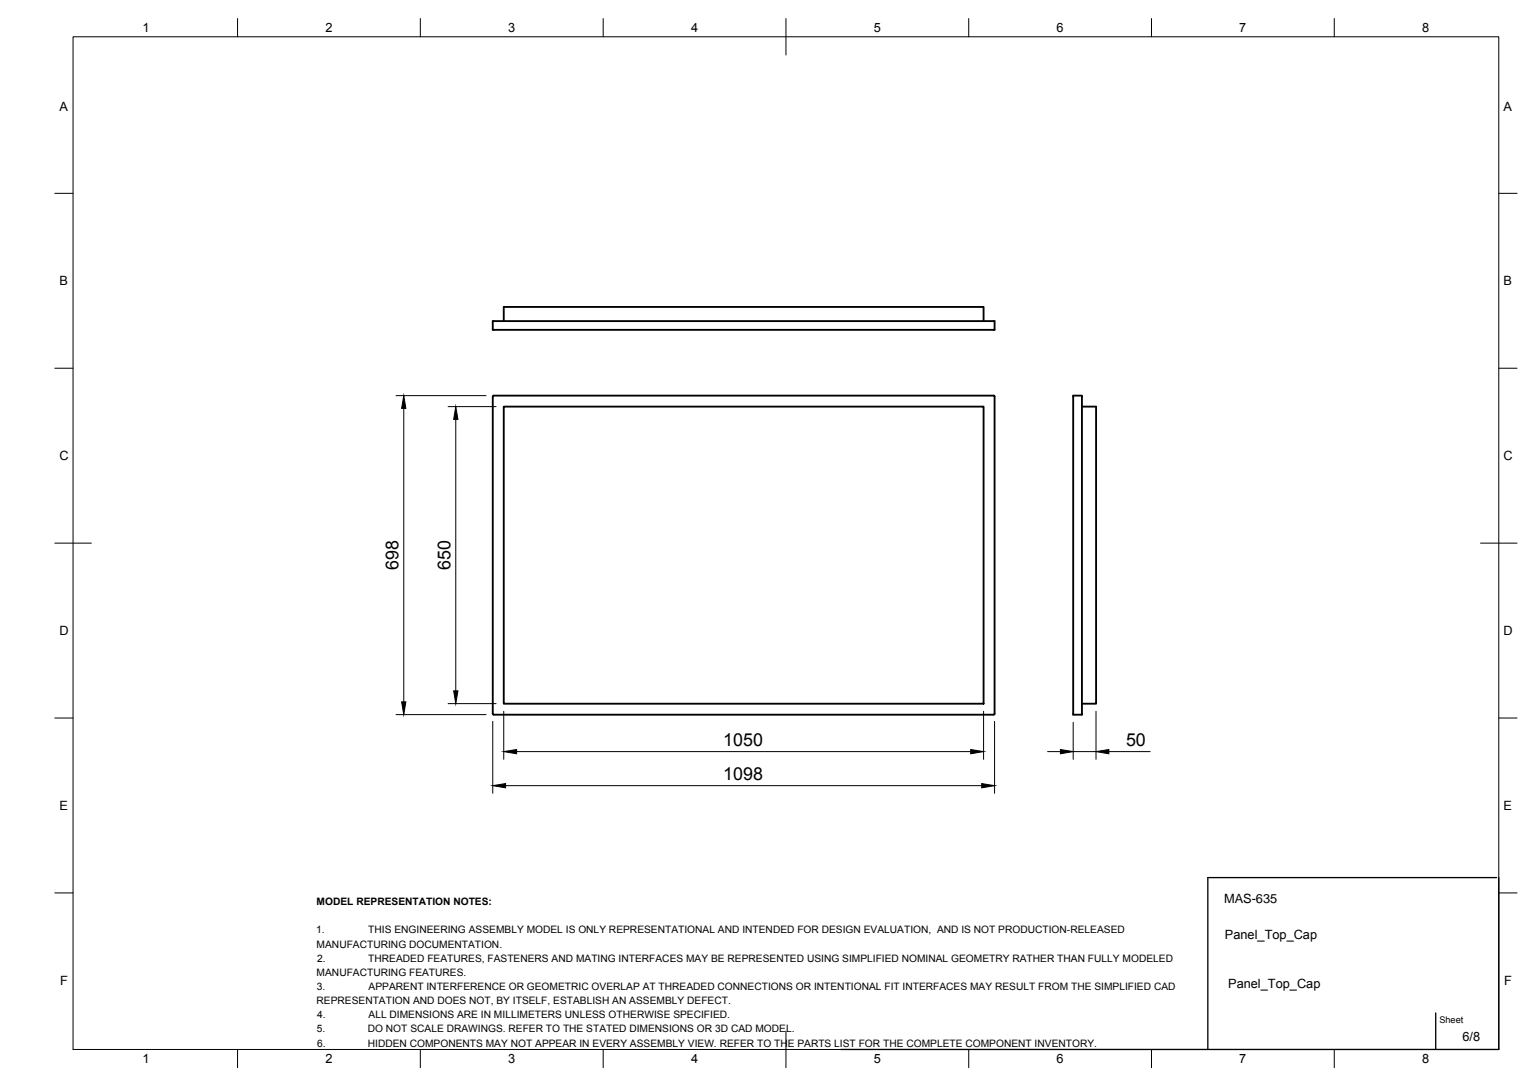
ISO-10303-21;
HEADER;
FILE_DESCRIPTION((''),'2;1');
FILE_NAME('Panel_Top_Cap.step','2026-10-09T12:34:24-07:00',(''),(''),'','','');
FILE_SCHEMA (('AUTOMOTIVE_DESIGN { 1 0 10303 214 3 1 1 }'));
ENDSEC;
DATA;
#10=MECHANICAL_DESIGN_GEOMETRIC_PRESENTATION_REPRESENTATION('',(#62),#3759);
#50=SHAPE_REPRESENTATION_RELATIONSHIP('SRR','None',#3791,#56) ;
#56=ADVANCED_BREP_SHAPE_REPRESENTATION('',(#68),#3756) ;
#62=STYLED_ITEM('',(#3827),#68) ;
#68=MANIFOLD_SOLID_BREP('Body1',#2266) ;
#83=CYLINDRICAL_SURFACE('',#2449,0.2) ;
#84=CYLINDRICAL_SURFACE('',#2450,0.2) ;
#85=CYLINDRICAL_SURFACE('',#2451,0.2) ;
#86=CYLINDRICAL_SURFACE('',#2452,0.2) ;
#111=CIRCLE('',#2440,0.2) ;
#112=CIRCLE('',#2441,0.2) ;
#113=CIRCLE('',#2442,0.2) ;
#114=CIRCLE('',#2443,0.2) ;
#115=CIRCLE('',#2445,0.2) ;
#116=CIRCLE('',#2446,0.2) ;
#117=CIRCLE('',#2447,0.2) ;
#118=CIRCLE('',#2448,0.2) ;
#132=FACE_BOUND('',#349,.T.) ;
#206=FACE_OUTER_BOUND('',#339,.T.) ;
#207=FACE_OUTER_BOUND('',#340,.T.) ;
#208=FACE_OUTER_BOUND('',#341,.T.) ;
#209=FACE_OUTER_BOUND('',#342,.T.) ;
#210=FACE_OUTER_BOUND('',#343,.T.) ;
#211=FACE_OUTER_BOUND('',#344,.T.) ;
#212=FACE_OUTER_BOUND('',#345,.T.) ;
#213=FACE_OUTER_BOUND('',#346,.T.) ;
#214=FACE_OUTER_BOUND('',#347,.T.) ;
#215=FACE_OUTER_BOUND('',#348,.T.) ;
#216=FACE_OUTER_BOUND('',#350,.T.) ;
#217=FACE_OUTER_BOUND('',#351,.T.) ;
#218=FACE_OUTER_BOUND('',#352,.T.) ;
#219=FACE_OUTER_BOUND('',#353,.T.) ;
#220=FACE_OUTER_BOUND('',#354,.T.) ;
#339=EDGE_LOOP('',(#1775,#1776,#1777,#1778)) ;
#340=EDGE_LOOP('',(#1779,#1780,#1781,#1782)) ;
#341=EDGE_LOOP('',(#1783,#1784,#1785,#1786)) ;
#342=EDGE_LOOP('',(#1787,#1788,#1789,#1790)) ;
#343=EDGE_LOOP('',(#1791,#1792,#1793,#1794)) ;
#344=EDGE_LOOP('',(#1795,#1796,#1797,#1798)) ;
#345=EDGE_LOOP('',(#1799,#1800,#1801,#1802)) ;
#346=EDGE_LOOP('',(#1803,#1804,#1805,#1806)) ;
#347=EDGE_LOOP('',(#1807,#1808,#1809,#1810)) ;
#348=EDGE_LOOP('',(#1811,#1812,#1813,#1814,#1815,#1816,#1817,#1818)) ;
#349=EDGE_LOOP('',(#1819,#1820,#1821,#1822)) ;
#350=EDGE_LOOP('',(#1823,#1824,#1825,#1826,#1827,#1828,#1829,#1830)) ;
#351=EDGE_LOOP('',(#1831,#1832,#1833,#1834)) ;
#352=EDGE_LOOP('',(#1835,#1836,#1837,#1838)) ;
#353=EDGE_LOOP('',(#1839,#1840,#1841,#1842)) ;
#354=EDGE_LOOP('',(#1843,#1844,#1845,#1846)) ;
#547=LINE('',#3461,#815) ;
#548=LINE('',#3463,#816) ;
#549=LINE('',#3465,#817) ;
#550=LINE('',#3466,#818) ;
#551=LINE('',#3469,#819) ;
#552=LINE('',#3471,#820) ;
#553=LINE('',#3472,#821) ;
#554=LINE('',#3475,#822) ;
#555=LINE('',#3477,#823) ;
#556=LINE('',#3478,#824) ;
#557=LINE('',#3480,#825) ;
#558=LINE('',#3481,#826) ;
#559=LINE('',#3486,#827) ;
#560=LINE('',#3488,#828) ;
#561=LINE('',#3490,#829) ;
#562=LINE('',#3491,#830) ;
#563=LINE('',#3495,#831) ;
#564=LINE('',#3497,#832) ;
#565=LINE('',#3499,#833) ;
#566=LINE('',#3500,#834) ;
#567=LINE('',#3504,#835) ;
#568=LINE('',#3506,#836) ;
#569=LINE('',#3508,#837) ;
#570=LINE('',#3509,#838) ;
#571=LINE('',#3513,#839) ;
#572=LINE('',#3515,#840) ;
#573=LINE('',#3517,#841) ;
#574=LINE('',#3518,#842) ;
#815=VECTOR('',#2838,100.) ;
#816=VECTOR('',#2839,100.) ;
#817=VECTOR('',#2840,100.) ;
#818=VECTOR('',#2841,100.) ;
#819=VECTOR('',#2844,100.) ;
#820=VECTOR('',#2845,100.) ;
#821=VECTOR('',#2846,100.) ;
#822=VECTOR('',#2849,100.) ;
#823=VECTOR('',#2850,100.) ;
#824=VECTOR('',#2851,100.) ;
#825=VECTOR('',#2854,100.) ;
#826=VECTOR('',#2855,100.) ;
#827=VECTOR('',#2860,100.) ;
#828=VECTOR('',#2861,100.) ;
#829=VECTOR('',#2862,100.) ;
#830=VECTOR('',#2863,100.) ;
#831=VECTOR('',#2866,100.) ;
#832=VECTOR('',#2867,100.) ;
#833=VECTOR('',#2868,100.) ;
#834=VECTOR('',#2869,100.) ;
#835=VECTOR('',#2872,100.) ;
#836=VECTOR('',#2873,100.) ;
#837=VECTOR('',#2874,100.) ;
#838=VECTOR('',#2875,100.) ;
#839=VECTOR('',#2878,100.) ;
#840=VECTOR('',#2879,100.) ;
#841=VECTOR('',#2880,100.) ;
#842=VECTOR('',#2881,100.) ;
#1051=VERTEX_POINT('',#3459) ;
#1052=VERTEX_POINT('',#3460) ;
#1053=VERTEX_POINT('',#3462) ;
#1054=VERTEX_POINT('',#3464) ;
#1055=VERTEX_POINT('',#3468) ;
#1056=VERTEX_POINT('',#3470) ;
#1057=VERTEX_POINT('',#3474) ;
#1058=VERTEX_POINT('',#3476) ;
#1059=VERTEX_POINT('',#3484) ;
#1060=VERTEX_POINT('',#3485) ;
#1061=VERTEX_POINT('',#3487) ;
#1062=VERTEX_POINT('',#3489) ;
#1063=VERTEX_POINT('',#3493) ;
#1064=VERTEX_POINT('',#3494) ;
#1065=VERTEX_POINT('',#3496) ;
#1066=VERTEX_POINT('',#3498) ;
#1067=VERTEX_POINT('',#3502) ;
#1068=VERTEX_POINT('',#3503) ;
#1069=VERTEX_POINT('',#3505) ;
#1070=VERTEX_POINT('',#3507) ;
#1071=VERTEX_POINT('',#3511) ;
#1072=VERTEX_POINT('',#3512) ;
#1073=VERTEX_POINT('',#3514) ;
#1074=VERTEX_POINT('',#3516) ;
#1307=EDGE_CURVE('',#1051,#1052,#547,.T.) ;
#1308=EDGE_CURVE('',#1053,#1051,#548,.T.) ;
#1309=EDGE_CURVE('',#1053,#1054,#549,.T.) ;
#1310=EDGE_CURVE('',#1054,#1052,#550,.T.) ;
#1311=EDGE_CURVE('',#1051,#1055,#551,.T.) ;
#1312=EDGE_CURVE('',#1056,#1055,#552,.T.) ;
#1313=EDGE_CURVE('',#1053,#1056,#553,.T.) ;
#1314=EDGE_CURVE('',#1055,#1057,#554,.T.) ;
#1315=EDGE_CURVE('',#1058,#1057,#555,.T.) ;
#1316=EDGE_CURVE('',#1056,#1058,#556,.T.) ;
#1317=EDGE_CURVE('',#1052,#1057,#557,.T.) ;
#1318=EDGE_CURVE('',#1054,#1058,#558,.T.) ;
#1319=EDGE_CURVE('',#1059,#1060,#559,.T.) ;
#1320=EDGE_CURVE('',#1059,#1061,#560,.T.) ;
#1321=EDGE_CURVE('',#1061,#1062,#561,.T.) ;
#1322=EDGE_CURVE('',#1062,#1060,#562,.T.) ;
#1323=EDGE_CURVE('',#1063,#1064,#563,.T.) ;
#1324=EDGE_CURVE('',#1064,#1065,#564,.T.) ;
#1325=EDGE_CURVE('',#1066,#1065,#565,.T.) ;
#1326=EDGE_CURVE('',#1066,#1063,#566,.T.) ;
#1327=EDGE_CURVE('',#1067,#1068,#567,.T.) ;
#1328=EDGE_CURVE('',#1067,#1069,#568,.T.) ;
#1329=EDGE_CURVE('',#1069,#1070,#569,.T.) ;
#1330=EDGE_CURVE('',#1070,#1068,#570,.T.) ;
#1331=EDGE_CURVE('',#1071,#1072,#571,.T.) ;
#1332=EDGE_CURVE('',#1071,#1073,#572,.T.) ;
#1333=EDGE_CURVE('',#1073,#1074,#573,.T.) ;
#1334=EDGE_CURVE('',#1074,#1072,#574,.T.) ;
#1335=EDGE_CURVE('',#1073,#1059,#111,.T.) ;
#1336=EDGE_CURVE('',#1060,#1066,#112,.T.) ;
#1337=EDGE_CURVE('',#1065,#1070,#113,.T.) ;
#1338=EDGE_CURVE('',#1069,#1074,#114,.T.) ;
#1339=EDGE_CURVE('',#1061,#1071,#115,.T.) ;
#1340=EDGE_CURVE('',#1072,#1067,#116,.T.) ;
#1341=EDGE_CURVE('',#1068,#1064,#117,.T.) ;
#1342=EDGE_CURVE('',#1063,#1062,#118,.T.) ;
#1775=ORIENTED_EDGE('',*,*,#1307,.F.) ;
#1776=ORIENTED_EDGE('',*,*,#1308,.F.) ;
#1777=ORIENTED_EDGE('',*,*,#1309,.T.) ;
#1778=ORIENTED_EDGE('',*,*,#1310,.T.) ;
#1779=ORIENTED_EDGE('',*,*,#1308,.T.) ;
#1780=ORIENTED_EDGE('',*,*,#1311,.T.) ;
#1781=ORIENTED_EDGE('',*,*,#1312,.F.) ;
#1782=ORIENTED_EDGE('',*,*,#1313,.F.) ;
#1783=ORIENTED_EDGE('',*,*,#1312,.T.) ;
#1784=ORIENTED_EDGE('',*,*,#1314,.T.) ;
#1785=ORIENTED_EDGE('',*,*,#1315,.F.) ;
#1786=ORIENTED_EDGE('',*,*,#1316,.F.) ;
#1787=ORIENTED_EDGE('',*,*,#1317,.F.) ;
#1788=ORIENTED_EDGE('',*,*,#1310,.F.) ;
#1789=ORIENTED_EDGE('',*,*,#1318,.T.) ;
#1790=ORIENTED_EDGE('',*,*,#1315,.T.) ;
#1791=ORIENTED_EDGE('',*,*,#1309,.F.) ;
#1792=ORIENTED_EDGE('',*,*,#1313,.T.) ;
#1793=ORIENTED_EDGE('',*,*,#1316,.T.) ;
#1794=ORIENTED_EDGE('',*,*,#1318,.F.) ;
#1795=ORIENTED_EDGE('',*,*,#1319,.F.) ;
#1796=ORIENTED_EDGE('',*,*,#1320,.T.) ;
#1797=ORIENTED_EDGE('',*,*,#1321,.T.) ;
#1798=ORIENTED_EDGE('',*,*,#1322,.T.) ;
#1799=ORIENTED_EDGE('',*,*,#1323,.T.) ;
#1800=ORIENTED_EDGE('',*,*,#1324,.T.) ;
#1801=ORIENTED_EDGE('',*,*,#1325,.F.) ;
#1802=ORIENTED_EDGE('',*,*,#1326,.T.) ;
#1803=ORIENTED_EDGE('',*,*,#1327,.F.) ;
#1804=ORIENTED_EDGE('',*,*,#1328,.T.) ;
#1805=ORIENTED_EDGE('',*,*,#1329,.T.) ;
#1806=ORIENTED_EDGE('',*,*,#1330,.T.) ;
#1807=ORIENTED_EDGE('',*,*,#1331,.F.) ;
#1808=ORIENTED_EDGE('',*,*,#1332,.T.) ;
#1809=ORIENTED_EDGE('',*,*,#1333,.T.) ;
#1810=ORIENTED_EDGE('',*,*,#1334,.T.) ;
#1811=ORIENTED_EDGE('',*,*,#1333,.F.) ;
#1812=ORIENTED_EDGE('',*,*,#1335,.T.) ;
#1813=ORIENTED_EDGE('',*,*,#1319,.T.) ;
#1814=ORIENTED_EDGE('',*,*,#1336,.T.) ;
#1815=ORIENTED_EDGE('',*,*,#1325,.T.) ;
#1816=ORIENTED_EDGE('',*,*,#1337,.T.) ;
#1817=ORIENTED_EDGE('',*,*,#1329,.F.) ;
#1818=ORIENTED_EDGE('',*,*,#1338,.T.) ;
#1819=ORIENTED_EDGE('',*,*,#1311,.F.) ;
#1820=ORIENTED_EDGE('',*,*,#1307,.T.) ;
#1821=ORIENTED_EDGE('',*,*,#1317,.T.) ;
#1822=ORIENTED_EDGE('',*,*,#1314,.F.) ;
#1823=ORIENTED_EDGE('',*,*,#1321,.F.) ;
#1824=ORIENTED_EDGE('',*,*,#1339,.T.) ;
#1825=ORIENTED_EDGE('',*,*,#1331,.T.) ;
#1826=ORIENTED_EDGE('',*,*,#1340,.T.) ;
#1827=ORIENTED_EDGE('',*,*,#1327,.T.) ;
#1828=ORIENTED_EDGE('',*,*,#1341,.T.) ;
#1829=ORIENTED_EDGE('',*,*,#1323,.F.) ;
#1830=ORIENTED_EDGE('',*,*,#1342,.T.) ;
#1831=ORIENTED_EDGE('',*,*,#1335,.F.) ;
#1832=ORIENTED_EDGE('',*,*,#1332,.F.) ;
#1833=ORIENTED_EDGE('',*,*,#1339,.F.) ;
#1834=ORIENTED_EDGE('',*,*,#1320,.F.) ;
#1835=ORIENTED_EDGE('',*,*,#1338,.F.) ;
#1836=ORIENTED_EDGE('',*,*,#1328,.F.) ;
#1837=ORIENTED_EDGE('',*,*,#1340,.F.) ;
#1838=ORIENTED_EDGE('',*,*,#1334,.F.) ;
#1839=ORIENTED_EDGE('',*,*,#1337,.F.) ;
#1840=ORIENTED_EDGE('',*,*,#1324,.F.) ;
#1841=ORIENTED_EDGE('',*,*,#1341,.F.) ;
#1842=ORIENTED_EDGE('',*,*,#1330,.F.) ;
#1843=ORIENTED_EDGE('',*,*,#1336,.F.) ;
#1844=ORIENTED_EDGE('',*,*,#1322,.F.) ;
#1845=ORIENTED_EDGE('',*,*,#1342,.F.) ;
#1846=ORIENTED_EDGE('',*,*,#1326,.F.) ;
#2092=PLANE('',#2430) ;
#2093=PLANE('',#2431) ;
#2094=PLANE('',#2432) ;
#2095=PLANE('',#2433) ;
#2096=PLANE('',#2434) ;
#2097=PLANE('',#2435) ;
#2098=PLANE('',#2436) ;
#2099=PLANE('',#2437) ;
#2100=PLANE('',#2438) ;
#2101=PLANE('',#2439) ;
#2102=PLANE('',#2444) ;
#2208=ADVANCED_FACE('',(#206),#2092,.T.) ;
#2209=ADVANCED_FACE('',(#207),#2093,.F.) ;
#2210=ADVANCED_FACE('',(#208),#2094,.F.) ;
#2211=ADVANCED_FACE('',(#209),#2095,.T.) ;
#2212=ADVANCED_FACE('',(#210),#2096,.F.) ;
#2213=ADVANCED_FACE('',(#211),#2097,.F.) ;
#2214=ADVANCED_FACE('',(#212),#2098,.F.) ;
#2215=ADVANCED_FACE('',(#213),#2099,.T.) ;
#2216=ADVANCED_FACE('',(#214),#2100,.T.) ;
#2217=ADVANCED_FACE('',(#215,#132),#2101,.T.) ;
#2218=ADVANCED_FACE('',(#216),#2102,.T.) ;
#2219=ADVANCED_FACE('',(#217),#83,.T.) ;
#2220=ADVANCED_FACE('',(#218),#84,.T.) ;
#2221=ADVANCED_FACE('',(#219),#85,.T.) ;
#2222=ADVANCED_FACE('',(#220),#86,.T.) ;
#2266=CLOSED_SHELL('',(#2208,#2209,#2210,#2211,#2212,#2213,#2214,#2215,
#2216,#2217,#2218,#2219,#2220,#2221,#2222)) ;
#2429=AXIS2_PLACEMENT_3D('',#3457,#2834,#2835) ;
#2430=AXIS2_PLACEMENT_3D('',#3458,#2836,#2837) ;
#2431=AXIS2_PLACEMENT_3D('',#3467,#2842,#2843) ;
#2432=AXIS2_PLACEMENT_3D('',#3473,#2847,#2848) ;
#2433=AXIS2_PLACEMENT_3D('',#3479,#2852,#2853) ;
#2434=AXIS2_PLACEMENT_3D('',#3482,#2856,#2857) ;
#2435=AXIS2_PLACEMENT_3D('',#3483,#2858,#2859) ;
#2436=AXIS2_PLACEMENT_3D('',#3492,#2864,#2865) ;
#2437=AXIS2_PLACEMENT_3D('',#3501,#2870,#2871) ;
#2438=AXIS2_PLACEMENT_3D('',#3510,#2876,#2877) ;
#2439=AXIS2_PLACEMENT_3D('',#3519,#2882,#2883) ;
#2440=AXIS2_PLACEMENT_3D('',#3520,#2884,#2885) ;
#2441=AXIS2_PLACEMENT_3D('',#3521,#2886,#2887) ;
#2442=AXIS2_PLACEMENT_3D('',#3522,#2888,#2889) ;
#2443=AXIS2_PLACEMENT_3D('',#3523,#2890,#2891) ;
#2444=AXIS2_PLACEMENT_3D('',#3524,#2892,#2893) ;
#2445=AXIS2_PLACEMENT_3D('',#3525,#2894,#2895) ;
#2446=AXIS2_PLACEMENT_3D('',#3526,#2896,#2897) ;
#2447=AXIS2_PLACEMENT_3D('',#3527,#2898,#2899) ;
#2448=AXIS2_PLACEMENT_3D('',#3528,#2900,#2901) ;
#2449=AXIS2_PLACEMENT_3D('',#3529,#2902,#2903) ;
#2450=AXIS2_PLACEMENT_3D('',#3530,#2904,#2905) ;
#2451=AXIS2_PLACEMENT_3D('',#3531,#2906,#2907) ;
#2452=AXIS2_PLACEMENT_3D('',#3532,#2908,#2909) ;
#2834=DIRECTION('axis',(0.,0.,1.)) ;
#2835=DIRECTION('refdir',(1.,0.,0.)) ;
#2836=DIRECTION('center_axis',(1.05735526154777E-16,-1.,0.)) ;
#2837=DIRECTION('ref_axis',(1.,1.05735526154777E-16,0.)) ;
#2838=DIRECTION('',(-1.,-1.05735526154777E-16,0.)) ;
#2839=DIRECTION('',(0.,0.,-1.)) ;
#2840=DIRECTION('',(-1.,-1.05735526154777E-16,0.)) ;
#2841=DIRECTION('',(0.,0.,-1.)) ;
#2842=DIRECTION('center_axis',(-1.,0.,0.)) ;
#2843=DIRECTION('ref_axis',(0.,0.,1.)) ;
#2844=DIRECTION('',(0.,1.,0.)) ;
#2845=DIRECTION('',(0.,0.,-1.)) ;
#2846=DIRECTION('',(0.,1.,0.)) ;
#2847=DIRECTION('center_axis',(1.05735526154777E-16,-1.,0.)) ;
#2848=DIRECTION('ref_axis',(1.,1.05735526154777E-16,0.)) ;
#2849=DIRECTION('',(-1.,-1.05735526154777E-16,0.)) ;
#2850=DIRECTION('',(0.,0.,-1.)) ;
#2851=DIRECTION('',(-1.,-1.05735526154777E-16,0.)) ;
#2852=DIRECTION('center_axis',(-1.,0.,0.)) ;
#2853=DIRECTION('ref_axis',(0.,0.,1.)) ;
#2854=DIRECTION('',(0.,1.,0.)) ;
#2855=DIRECTION('',(0.,1.,0.)) ;
#2856=DIRECTION('center_axis',(0.,0.,-1.)) ;
#2857=DIRECTION('ref_axis',(-1.,0.,0.)) ;
#2858=DIRECTION('center_axis',(-1.,0.,0.)) ;
#2859=DIRECTION('ref_axis',(0.,0.,1.)) ;
#2860=DIRECTION('',(0.,1.,0.)) ;
#2861=DIRECTION('',(0.,0.,-1.)) ;
#2862=DIRECTION('',(0.,1.,0.)) ;
#2863=DIRECTION('',(0.,0.,1.)) ;
#2864=DIRECTION('center_axis',(1.01113208071508E-16,-1.,0.)) ;
#2865=DIRECTION('ref_axis',(1.,1.01113208071508E-16,0.)) ;
#2866=DIRECTION('',(-1.,-1.01113208071508E-16,0.)) ;
#2867=DIRECTION('',(0.,0.,1.)) ;
#2868=DIRECTION('',(-1.,-1.01113208071508E-16,0.)) ;
#2869=DIRECTION('',(0.,0.,-1.)) ;
#2870=DIRECTION('center_axis',(-1.,0.,0.)) ;
#2871=DIRECTION('ref_axis',(0.,0.,1.)) ;
#2872=DIRECTION('',(0.,1.,0.)) ;
#2873=DIRECTION('',(0.,0.,1.)) ;
#2874=DIRECTION('',(0.,1.,0.)) ;
#2875=DIRECTION('',(0.,0.,-1.)) ;
#2876=DIRECTION('center_axis',(1.51669812107262E-16,-1.,0.)) ;
#2877=DIRECTION('ref_axis',(1.,1.51669812107262E-16,0.)) ;
#2878=DIRECTION('',(-1.,-1.51669812107262E-16,0.)) ;
#2879=DIRECTION('',(0.,0.,1.)) ;
#2880=DIRECTION('',(-1.,-1.51669812107262E-16,0.)) ;
#2881=DIRECTION('',(0.,0.,-1.)) ;
#2882=DIRECTION('center_axis',(0.,0.,1.)) ;
#2883=DIRECTION('ref_axis',(1.,0.,0.)) ;
#2884=DIRECTION('center_axis',(0.,0.,1.)) ;
#2885=DIRECTION('ref_axis',(1.,0.,0.)) ;
#2886=DIRECTION('center_axis',(0.,0.,1.)) ;
#2887=DIRECTION('ref_axis',(1.,0.,0.)) ;
#2888=DIRECTION('center_axis',(0.,0.,1.)) ;
#2889=DIRECTION('ref_axis',(1.,0.,0.)) ;
#2890=DIRECTION('center_axis',(0.,0.,1.)) ;
#2891=DIRECTION('ref_axis',(1.,0.,0.)) ;
#2892=DIRECTION('center_axis',(0.,0.,-1.)) ;
#2893=DIRECTION('ref_axis',(-1.,0.,0.)) ;
#2894=DIRECTION('center_axis',(0.,0.,-1.)) ;
#2895=DIRECTION('ref_axis',(-1.,0.,0.)) ;
#2896=DIRECTION('center_axis',(0.,0.,-1.)) ;
#2897=DIRECTION('ref_axis',(-1.,0.,0.)) ;
#2898=DIRECTION('center_axis',(0.,0.,-1.)) ;
#2899=DIRECTION('ref_axis',(-1.,0.,0.)) ;
#2900=DIRECTION('center_axis',(0.,0.,-1.)) ;
#2901=DIRECTION('ref_axis',(-1.,0.,0.)) ;
#2902=DIRECTION('center_axis',(0.,0.,1.)) ;
#2903=DIRECTION('ref_axis',(1.,0.,0.)) ;
#2904=DIRECTION('center_axis',(0.,0.,-1.)) ;
#2905=DIRECTION('ref_axis',(-1.,0.,0.)) ;
#2906=DIRECTION('center_axis',(0.,0.,1.)) ;
#2907=DIRECTION('ref_axis',(1.,0.,0.)) ;
#2908=DIRECTION('center_axis',(0.,0.,-1.)) ;
#2909=DIRECTION('ref_axis',(-1.,0.,0.)) ;
#3457=CARTESIAN_POINT('',(0.,0.,0.)) ;
#3458=CARTESIAN_POINT('Origin',(52.5,-32.5,5.)) ;
#3459=CARTESIAN_POINT('',(52.5,-32.5,1.9)) ;
#3460=CARTESIAN_POINT('',(-52.5,-32.5,1.9)) ;
#3461=CARTESIAN_POINT('',(52.5,-32.5,1.9)) ;
#3462=CARTESIAN_POINT('',(52.5,-32.5,5.)) ;
#3463=CARTESIAN_POINT('',(52.5,-32.5,5.)) ;
#3464=CARTESIAN_POINT('',(-52.5,-32.5,5.)) ;
#3465=CARTESIAN_POINT('',(52.5,-32.5,5.)) ;
#3466=CARTESIAN_POINT('',(-52.5,-32.5,5.)) ;
#3467=CARTESIAN_POINT('Origin',(52.5,-32.5,5.)) ;
#3468=CARTESIAN_POINT('',(52.5,32.5,1.9)) ;
#3469=CARTESIAN_POINT('',(52.5,-32.5,1.9)) ;
#3470=CARTESIAN_POINT('',(52.5,32.5,5.)) ;
#3471=CARTESIAN_POINT('',(52.5,32.5,5.)) ;
#3472=CARTESIAN_POINT('',(52.5,-32.5,5.)) ;
#3473=CARTESIAN_POINT('Origin',(52.5,32.5,5.)) ;
#3474=CARTESIAN_POINT('',(-52.5,32.5,1.9)) ;
#3475=CARTESIAN_POINT('',(52.5,32.5,1.9)) ;
#3476=CARTESIAN_POINT('',(-52.5,32.5,5.)) ;
#3477=CARTESIAN_POINT('',(-52.5,32.5,5.)) ;
#3478=CARTESIAN_POINT('',(52.5,32.5,5.)) ;
#3479=CARTESIAN_POINT('Origin',(-52.5,-32.5,5.)) ;
#3480=CARTESIAN_POINT('',(-52.5,-32.5,1.9)) ;
#3481=CARTESIAN_POINT('',(-52.5,-32.5,5.)) ;
#3482=CARTESIAN_POINT('Origin',(0.,0.,5.)) ;
#3483=CARTESIAN_POINT('Origin',(54.9,-34.9,1.9)) ;
#3484=CARTESIAN_POINT('',(54.9,-34.7,1.9)) ;
#3485=CARTESIAN_POINT('',(54.9,34.7,1.9)) ;
#3486=CARTESIAN_POINT('',(54.9,-34.9,1.9)) ;
#3487=CARTESIAN_POINT('',(54.9,-34.7,0.)) ;
#3488=CARTESIAN_POINT('',(54.9,-34.7,0.)) ;
#3489=CARTESIAN_POINT('',(54.9,34.7,0.)) ;
#3490=CARTESIAN_POINT('',(54.9,-34.9,0.)) ;
#3491=CARTESIAN_POINT('',(54.9,34.7,1.9)) ;
#3492=CARTESIAN_POINT('Origin',(54.9,34.9,1.9)) ;
#3493=CARTESIAN_POINT('',(54.7,34.9,0.)) ;
#3494=CARTESIAN_POINT('',(-54.7,34.9,0.)) ;
#3495=CARTESIAN_POINT('',(54.9,34.9,0.)) ;
#3496=CARTESIAN_POINT('',(-54.7,34.9,1.9)) ;
#3497=CARTESIAN_POINT('',(-54.7,34.9,1.9)) ;
#3498=CARTESIAN_POINT('',(54.7,34.9,1.9)) ;
#3499=CARTESIAN_POINT('',(54.9,34.9,1.9)) ;
#3500=CARTESIAN_POINT('',(54.7,34.9,1.9)) ;
#3501=CARTESIAN_POINT('Origin',(-54.9,-34.9,1.9)) ;
#3502=CARTESIAN_POINT('',(-54.9,-34.7,0.)) ;
#3503=CARTESIAN_POINT('',(-54.9,34.7,0.)) ;
#3504=CARTESIAN_POINT('',(-54.9,-34.9,0.)) ;
#3505=CARTESIAN_POINT('',(-54.9,-34.7,1.9)) ;
#3506=CARTESIAN_POINT('',(-54.9,-34.7,1.9)) ;
#3507=CARTESIAN_POINT('',(-54.9,34.7,1.9)) ;
#3508=CARTESIAN_POINT('',(-54.9,-34.9,1.9)) ;
#3509=CARTESIAN_POINT('',(-54.9,34.7,0.)) ;
#3510=CARTESIAN_POINT('Origin',(54.9,-34.9,1.9)) ;
#3511=CARTESIAN_POINT('',(54.7,-34.9,0.)) ;
#3512=CARTESIAN_POINT('',(-54.7,-34.9,0.)) ;
#3513=CARTESIAN_POINT('',(54.9,-34.9,0.)) ;
#3514=CARTESIAN_POINT('',(54.7,-34.9,1.9)) ;
#3515=CARTESIAN_POINT('',(54.7,-34.9,1.9)) ;
#3516=CARTESIAN_POINT('',(-54.7,-34.9,1.9)) ;
#3517=CARTESIAN_POINT('',(54.9,-34.9,1.9)) ;
#3518=CARTESIAN_POINT('',(-54.7,-34.9,1.9)) ;
#3519=CARTESIAN_POINT('Origin',(0.,0.,1.9)) ;
#3520=CARTESIAN_POINT('Origin',(54.7,-34.7,1.9)) ;
#3521=CARTESIAN_POINT('Origin',(54.7,34.7,1.9)) ;
#3522=CARTESIAN_POINT('Origin',(-54.7,34.7,1.9)) ;
#3523=CARTESIAN_POINT('Origin',(-54.7,-34.7,1.9)) ;
#3524=CARTESIAN_POINT('Origin',(0.,0.,0.)) ;
#3525=CARTESIAN_POINT('Origin',(54.7,-34.7,0.)) ;
#3526=CARTESIAN_POINT('Origin',(-54.7,-34.7,0.)) ;
#3527=CARTESIAN_POINT('Origin',(-54.7,34.7,0.)) ;
#3528=CARTESIAN_POINT('Origin',(54.7,34.7,0.)) ;
#3529=CARTESIAN_POINT('Origin',(54.7,-34.7,1.9)) ;
#3530=CARTESIAN_POINT('Origin',(-54.7,-34.7,1.9)) ;
#3531=CARTESIAN_POINT('Origin',(-54.7,34.7,1.9)) ;
#3532=CARTESIAN_POINT('Origin',(54.7,34.7,1.9)) ;
#3748=UNCERTAINTY_MEASURE_WITH_UNIT(LENGTH_MEASURE(0.001),#3760,
'DISTANCE_ACCURACY_VALUE',
'Maximum model space distance between geometric entities at asserted c
onnectivities') ;
#3751=UNCERTAINTY_MEASURE_WITH_UNIT(LENGTH_MEASURE(0.001),#3760,
'DISTANCE_ACCURACY_VALUE',
'Maximum model space distance between geometric entities at asserted c
onnectivities') ;
#3756=(
GEOMETRIC_REPRESENTATION_CONTEXT(3)
GLOBAL_UNCERTAINTY_ASSIGNED_CONTEXT((#3748))
GLOBAL_UNIT_ASSIGNED_CONTEXT((#3760,#3762,#3763))
REPRESENTATION_CONTEXT('','3D')
) ;
#3759=(
GEOMETRIC_REPRESENTATION_CONTEXT(3)
GLOBAL_UNCERTAINTY_ASSIGNED_CONTEXT((#3751))
GLOBAL_UNIT_ASSIGNED_CONTEXT((#3760,#3762,#3763))
REPRESENTATION_CONTEXT('','3D')
) ;
#3760=(
LENGTH_UNIT()
NAMED_UNIT(*)
SI_UNIT(.CENTI.,.METRE.)
) ;
#3762=(
NAMED_UNIT(*)
PLANE_ANGLE_UNIT()
SI_UNIT($,.RADIAN.)
) ;
#3763=(
NAMED_UNIT(*)
SI_UNIT($,.STERADIAN.)
SOLID_ANGLE_UNIT()
) ;
#3768=SHAPE_DEFINITION_REPRESENTATION(#3775,#3791) ;
#3775=PRODUCT_DEFINITION_SHAPE('',$,#3799) ;
#3791=SHAPE_REPRESENTATION('',(#2429),#3756) ;
#3794=PRODUCT_DEFINITION_CONTEXT('part definition',#3817,'design') ;
#3799=PRODUCT_DEFINITION('Panel_Top_Cap','Panel_Top_Cap',#3806,
#3794) ;
#3806=PRODUCT_DEFINITION_FORMATION('',$,#3823) ;
#3817=APPLICATION_CONTEXT(
'Core Data for Automotive Mechanical Design Process') ;
#3818=PRODUCT_CONTEXT('part definition',#3817,'mechanical') ;
#3823=PRODUCT('Panel_Top_Cap','Panel_Top_Cap',$,(#3818)) ;
#3827=PRESENTATION_STYLE_ASSIGNMENT((#3829)) ;
#3829=SURFACE_STYLE_USAGE(.BOTH.,#3831) ;
#3831=SURFACE_SIDE_STYLE('',(#3833)) ;
#3833=SURFACE_STYLE_FILL_AREA(#3835) ;
#3835=FILL_AREA_STYLE('Opaque(179,179,179)',(#3837)) ;
#3837=FILL_AREA_STYLE_COLOUR('Opaque(179,179,179)',#3839) ;
#3839=COLOUR_RGB('Opaque(179,179,179)', 0.09019608, 0.27058824, 0.51372549) ;
ENDSEC;
END-ISO-10303-21;
